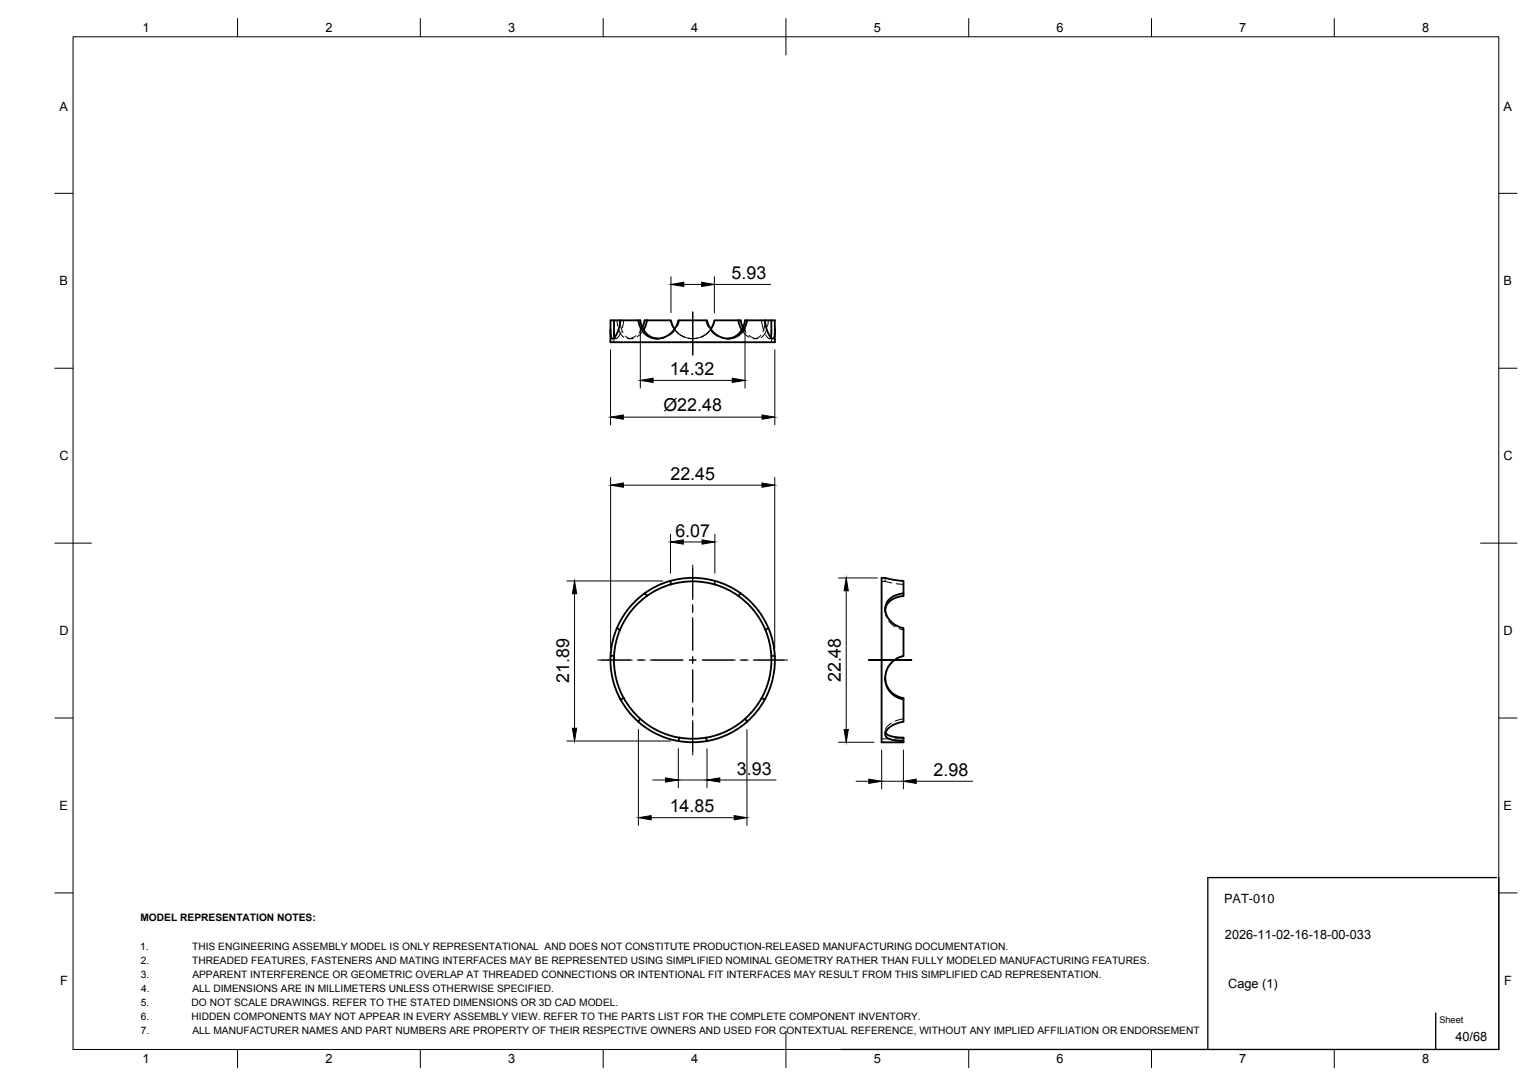
ISO-10303-21;
HEADER;
/* Generated by software containing ST-Developer
 * from STEP Tools, Inc. (www.steptools.com) 
 */

FILE_DESCRIPTION(
/* description */ ('Belt conveyor head drive unit'),
/* implementation_level */ '2;1');

FILE_NAME(
/* name */ 'Cage (1).step',
/* time_stamp */ '2026-10-28T03:26:19-07:00',
/* author */ (''),
/* organization */ (''),
/* preprocessor_version */ 'ST-DEVELOPER v20.2',
/* originating_system */ 'Autodesk Translation Framework v15.17.0.0',
/* authorisation */ '');

FILE_SCHEMA (('AUTOMOTIVE_DESIGN { 1 0 10303 214 3 1 1 }'));
ENDSEC;

DATA;
#10=MECHANICAL_DESIGN_GEOMETRIC_PRESENTATION_REPRESENTATION('',(#897),#27069);
#539=B_SPLINE_CURVE_WITH_KNOTS('',3,(#23163,#23164,#23165,#23166,#23167,
#23168,#23169,#23170,#23171,#23172,#23173,#23174,#23175,#23176,#23177,#23178,
#23179,#23180,#23181,#23182,#23183,#23184),.UNSPECIFIED.,.F.,.F.,(4,2,2,
2,2,2,2,2,2,2,4),(0.0591825211272536,0.157966726598481,0.236950089897721,
0.315933453196962,0.391576304923761,0.46721915665056,0.54286200837736,0.618504860104159,
0.697488223403399,0.77647158670264,0.875255792173867),.UNSPECIFIED.);
#540=B_SPLINE_CURVE_WITH_KNOTS('',3,(#23188,#23189,#23190,#23191,#23192,
#23193,#23194,#23195,#23196,#23197,#23198,#23199,#23200,#23201,#23202,#23203,
#23204,#23205,#23206,#23207,#23208,#23209),.UNSPECIFIED.,.F.,.F.,(4,2,2,
2,2,2,2,2,2,2,4),(0.0581119756758434,0.106553146291161,0.213106292582322,
0.30849933801665,0.386091982889075,0.4636846277615,0.541277272633925,0.61886991750635,
0.714262962940678,0.820816109231839,0.869257279847157),.UNSPECIFIED.);
#541=B_SPLINE_CURVE_WITH_KNOTS('',3,(#23215,#23216,#23217,#23218,#23219,
#23220,#23221,#23222,#23223,#23224,#23225,#23226,#23227,#23228,#23229,#23230,
#23231,#23232,#23233,#23234,#23235,#23236),.UNSPECIFIED.,.F.,.F.,(4,2,2,
2,2,2,2,2,2,2,4),(0.0581119756758434,0.106553146291161,0.213106292582322,
0.30849933801665,0.386091982889075,0.4636846277615,0.541277272633925,0.61886991750635,
0.714262962940679,0.820816109231839,0.869257279847157),.UNSPECIFIED.);
#542=B_SPLINE_CURVE_WITH_KNOTS('',3,(#23240,#23241,#23242,#23243,#23244,
#23245,#23246,#23247,#23248,#23249,#23250,#23251,#23252,#23253,#23254,#23255,
#23256,#23257,#23258,#23259,#23260,#23261),.UNSPECIFIED.,.F.,.F.,(4,2,2,
2,2,2,2,2,2,2,4),(0.0581119756758433,0.106553146291161,0.213106292582322,
0.308499338016649,0.386091982889075,0.4636846277615,0.541277272633925,0.61886991750635,
0.714262962940678,0.820816109231839,0.869257279847157),.UNSPECIFIED.);
#543=B_SPLINE_CURVE_WITH_KNOTS('',3,(#23270,#23271,#23272,#23273,#23274,
#23275,#23276,#23277,#23278,#23279,#23280,#23281,#23282,#23283,#23284,#23285,
#23286,#23287,#23288,#23289,#23290,#23291),.UNSPECIFIED.,.F.,.F.,(4,2,2,
2,2,2,2,2,2,2,4),(0.0581119756758433,0.106553146291161,0.213106292582322,
0.30849933801665,0.386091982889075,0.4636846277615,0.541277272633925,0.61886991750635,
0.714262962940678,0.820816109231839,0.869257279847157),.UNSPECIFIED.);
#544=B_SPLINE_CURVE_WITH_KNOTS('',3,(#23295,#23296,#23297,#23298,#23299,
#23300,#23301,#23302,#23303,#23304,#23305,#23306,#23307,#23308,#23309,#23310,
#23311,#23312,#23313,#23314,#23315,#23316),.UNSPECIFIED.,.F.,.F.,(4,2,2,
2,2,2,2,2,2,2,4),(0.0581119756758434,0.106553146291161,0.213106292582322,
0.30849933801665,0.386091982889075,0.4636846277615,0.541277272633925,0.61886991750635,
0.714262962940678,0.820816109231839,0.869257279847157),.UNSPECIFIED.);
#545=B_SPLINE_CURVE_WITH_KNOTS('',3,(#23320,#23321,#23322,#23323,#23324,
#23325,#23326,#23327,#23328,#23329,#23330,#23331,#23332,#23333,#23334,#23335,
#23336,#23337,#23338,#23339,#23340,#23341),.UNSPECIFIED.,.F.,.F.,(4,2,2,
2,2,2,2,2,2,2,4),(0.0581119756758434,0.106553146291161,0.213106292582322,
0.30849933801665,0.386091982889075,0.4636846277615,0.541277272633925,0.61886991750635,
0.714262962940678,0.820816109231839,0.869257279847157),.UNSPECIFIED.);
#546=B_SPLINE_CURVE_WITH_KNOTS('',3,(#23345,#23346,#23347,#23348,#23349,
#23350,#23351,#23352,#23353,#23354,#23355,#23356,#23357,#23358,#23359,#23360,
#23361,#23362,#23363,#23364,#23365,#23366),.UNSPECIFIED.,.F.,.F.,(4,2,2,
2,2,2,2,2,2,2,4),(0.0581119756758433,0.106553146291161,0.213106292582322,
0.30849933801665,0.386091982889075,0.4636846277615,0.541277272633925,0.61886991750635,
0.714262962940678,0.820816109231839,0.869257279847157),.UNSPECIFIED.);
#547=B_SPLINE_CURVE_WITH_KNOTS('',3,(#23374,#23375,#23376,#23377,#23378,
#23379,#23380,#23381,#23382,#23383,#23384,#23385,#23386,#23387,#23388,#23389,
#23390,#23391,#23392,#23393,#23394,#23395),.UNSPECIFIED.,.F.,.F.,(4,2,2,
2,2,2,2,2,2,2,4),(0.0591825211272536,0.157966726598481,0.236950089897721,
0.315933453196962,0.391576304923761,0.467219156650561,0.54286200837736,
0.618504860104159,0.697488223403399,0.77647158670264,0.875255792173867),
 .UNSPECIFIED.);
#548=B_SPLINE_CURVE_WITH_KNOTS('',3,(#23403,#23404,#23405,#23406,#23407,
#23408,#23409,#23410,#23411,#23412,#23413,#23414,#23415,#23416,#23417,#23418,
#23419,#23420,#23421,#23422,#23423,#23424),.UNSPECIFIED.,.F.,.F.,(4,2,2,
2,2,2,2,2,2,2,4),(0.0591825211272536,0.157966726598481,0.236950089897722,
0.315933453196962,0.391576304923761,0.467219156650561,0.54286200837736,
0.618504860104159,0.697488223403399,0.77647158670264,0.875255792173867),
 .UNSPECIFIED.);
#549=B_SPLINE_CURVE_WITH_KNOTS('',3,(#23434,#23435,#23436,#23437,#23438,
#23439,#23440,#23441,#23442,#23443,#23444,#23445,#23446,#23447,#23448,#23449,
#23450,#23451,#23452,#23453,#23454,#23455),.UNSPECIFIED.,.F.,.F.,(4,2,2,
2,2,2,2,2,2,2,4),(0.0591825211272536,0.157966726598481,0.236950089897721,
0.315933453196962,0.391576304923761,0.46721915665056,0.54286200837736,0.618504860104159,
0.697488223403399,0.77647158670264,0.875255792173867),.UNSPECIFIED.);
#550=B_SPLINE_CURVE_WITH_KNOTS('',3,(#23463,#23464,#23465,#23466,#23467,
#23468,#23469,#23470,#23471,#23472,#23473,#23474,#23475,#23476,#23477,#23478,
#23479,#23480,#23481,#23482,#23483,#23484),.UNSPECIFIED.,.F.,.F.,(4,2,2,
2,2,2,2,2,2,2,4),(0.0591825211272536,0.157966726598481,0.236950089897721,
0.315933453196962,0.391576304923761,0.46721915665056,0.542862008377359,
0.618504860104159,0.697488223403399,0.776471586702639,0.875255792173867),
 .UNSPECIFIED.);
#551=B_SPLINE_CURVE_WITH_KNOTS('',3,(#23492,#23493,#23494,#23495,#23496,
#23497,#23498,#23499,#23500,#23501,#23502,#23503,#23504,#23505,#23506,#23507,
#23508,#23509,#23510,#23511,#23512,#23513),.UNSPECIFIED.,.F.,.F.,(4,2,2,
2,2,2,2,2,2,2,4),(0.0591825211272536,0.157966726598481,0.236950089897721,
0.315933453196962,0.391576304923761,0.46721915665056,0.54286200837736,0.618504860104159,
0.697488223403399,0.77647158670264,0.875255792173867),.UNSPECIFIED.);
#552=B_SPLINE_CURVE_WITH_KNOTS('',3,(#23522,#23523,#23524,#23525,#23526,
#23527,#23528,#23529,#23530,#23531,#23532,#23533,#23534,#23535,#23536,#23537,
#23538,#23539,#23540,#23541,#23542,#23543),.UNSPECIFIED.,.F.,.F.,(4,2,2,
2,2,2,2,2,2,2,4),(0.0591825211272536,0.157966726598481,0.236950089897721,
0.315933453196962,0.391576304923761,0.46721915665056,0.542862008377359,
0.618504860104159,0.697488223403399,0.776471586702639,0.875255792173867),
 .UNSPECIFIED.);
#668=SPHERICAL_SURFACE('',#15410,0.309556);
#669=SPHERICAL_SURFACE('',#15426,0.309556);
#670=SPHERICAL_SURFACE('',#15431,0.309556);
#671=SPHERICAL_SURFACE('',#15437,0.309556);
#672=SPHERICAL_SURFACE('',#15442,0.309556);
#673=SPHERICAL_SURFACE('',#15447,0.309556);
#674=SPHERICAL_SURFACE('',#15455,0.309556);
#745=SHAPE_REPRESENTATION_RELATIONSHIP('SRR','None',#27391,#814);
#814=ADVANCED_BREP_SHAPE_REPRESENTATION('',(#981),#27033);
#897=STYLED_ITEM('',(#27797),#981);
#981=MANIFOLD_SOLID_BREP('Continuous crown cage',#13763);
#1166=FACE_BOUND('',#2998,.T.);
#1470=PLANE('',#15423);
#1471=PLANE('',#15428);
#1472=PLANE('',#15433);
#1473=PLANE('',#15439);
#1474=PLANE('',#15444);
#1475=PLANE('',#15453);
#1476=PLANE('',#15457);
#1477=PLANE('',#15458);
#2028=FACE_OUTER_BOUND('',#2982,.T.);
#2029=FACE_OUTER_BOUND('',#2983,.T.);
#2030=FACE_OUTER_BOUND('',#2984,.T.);
#2031=FACE_OUTER_BOUND('',#2985,.T.);
#2032=FACE_OUTER_BOUND('',#2986,.T.);
#2033=FACE_OUTER_BOUND('',#2987,.T.);
#2034=FACE_OUTER_BOUND('',#2988,.T.);
#2035=FACE_OUTER_BOUND('',#2989,.T.);
#2036=FACE_OUTER_BOUND('',#2990,.T.);
#2037=FACE_OUTER_BOUND('',#2991,.T.);
#2038=FACE_OUTER_BOUND('',#2992,.T.);
#2039=FACE_OUTER_BOUND('',#2993,.T.);
#2040=FACE_OUTER_BOUND('',#2994,.T.);
#2041=FACE_OUTER_BOUND('',#2995,.T.);
#2042=FACE_OUTER_BOUND('',#2996,.T.);
#2043=FACE_OUTER_BOUND('',#2997,.T.);
#2044=FACE_OUTER_BOUND('',#2999,.T.);
#2982=EDGE_LOOP('',(#10632,#10633,#10634,#10635));
#2983=EDGE_LOOP('',(#10636,#10637,#10638,#10639,#10640,#10641,#10642,#10643,
#10644,#10645,#10646,#10647,#10648,#10649,#10650,#10651,#10652,#10653));
#2984=EDGE_LOOP('',(#10654,#10655,#10656,#10657));
#2985=EDGE_LOOP('',(#10658,#10659,#10660,#10661));
#2986=EDGE_LOOP('',(#10662,#10663,#10664,#10665));
#2987=EDGE_LOOP('',(#10666,#10667,#10668,#10669));
#2988=EDGE_LOOP('',(#10670,#10671,#10672,#10673,#10674,#10675));
#2989=EDGE_LOOP('',(#10676,#10677,#10678,#10679));
#2990=EDGE_LOOP('',(#10680,#10681,#10682,#10683));
#2991=EDGE_LOOP('',(#10684,#10685,#10686,#10687));
#2992=EDGE_LOOP('',(#10688,#10689,#10690,#10691));
#2993=EDGE_LOOP('',(#10692,#10693,#10694,#10695));
#2994=EDGE_LOOP('',(#10696,#10697,#10698,#10699,#10700,#10701,#10702,#10703,
#10704,#10705,#10706,#10707,#10708,#10709,#10710,#10711,#10712,#10713));
#2995=EDGE_LOOP('',(#10714,#10715,#10716,#10717));
#2996=EDGE_LOOP('',(#10718,#10719,#10720,#10721));
#2997=EDGE_LOOP('',(#10722));
#2998=EDGE_LOOP('',(#10723));
#2999=EDGE_LOOP('',(#10724,#10725,#10726,#10727));
#3910=LINE('',#23265,#4702);
#3911=LINE('',#23518,#4703);
#4702=VECTOR('',#18556,1.123812);
#4703=VECTOR('',#18625,1.076188);
#5489=CIRCLE('',#15411,0.303778037777585);
#5490=CIRCLE('',#15412,0.303778037777585);
#5491=CIRCLE('',#15414,1.123812);
#5492=CIRCLE('',#15415,1.123812);
#5493=CIRCLE('',#15416,1.123812);
#5494=CIRCLE('',#15417,1.123812);
#5495=CIRCLE('',#15418,1.123812);
#5496=CIRCLE('',#15419,1.123812);
#5497=CIRCLE('',#15420,1.123812);
#5498=CIRCLE('',#15421,1.123812);
#5499=CIRCLE('',#15422,1.123812);
#5500=CIRCLE('',#15424,1.076188);
#5501=CIRCLE('',#15425,0.303778037777585);
#5502=CIRCLE('',#15427,0.303778037777585);
#5503=CIRCLE('',#15429,1.076188);
#5504=CIRCLE('',#15430,0.303778037777585);
#5505=CIRCLE('',#15432,0.303778037777585);
#5506=CIRCLE('',#15434,1.076188);
#5507=CIRCLE('',#15435,1.076188);
#5508=CIRCLE('',#15436,0.303778037777585);
#5509=CIRCLE('',#15438,0.303778037777585);
#5510=CIRCLE('',#15440,1.076188);
#5511=CIRCLE('',#15441,0.303778037777585);
#5512=CIRCLE('',#15443,0.303778037777585);
#5513=CIRCLE('',#15445,1.076188);
#5514=CIRCLE('',#15446,0.303778037777585);
#5515=CIRCLE('',#15448,0.303778037777585);
#5516=CIRCLE('',#15450,1.076188);
#5517=CIRCLE('',#15451,1.076188);
#5518=CIRCLE('',#15452,1.076188);
#5519=CIRCLE('',#15454,0.303778037777585);
#5520=CIRCLE('',#15456,0.303778037777585);
#6527=VERTEX_POINT('',#23161);
#6528=VERTEX_POINT('',#23162);
#6529=VERTEX_POINT('',#23185);
#6530=VERTEX_POINT('',#23187);
#6531=VERTEX_POINT('',#23212);
#6532=VERTEX_POINT('',#23214);
#6533=VERTEX_POINT('',#23237);
#6534=VERTEX_POINT('',#23239);
#6535=VERTEX_POINT('',#23262);
#6536=VERTEX_POINT('',#23264);
#6537=VERTEX_POINT('',#23267);
#6538=VERTEX_POINT('',#23269);
#6539=VERTEX_POINT('',#23292);
#6540=VERTEX_POINT('',#23294);
#6541=VERTEX_POINT('',#23317);
#6542=VERTEX_POINT('',#23319);
#6543=VERTEX_POINT('',#23342);
#6544=VERTEX_POINT('',#23344);
#6545=VERTEX_POINT('',#23369);
#6546=VERTEX_POINT('',#23373);
#6547=VERTEX_POINT('',#23398);
#6548=VERTEX_POINT('',#23402);
#6549=VERTEX_POINT('',#23427);
#6550=VERTEX_POINT('',#23429);
#6551=VERTEX_POINT('',#23433);
#6552=VERTEX_POINT('',#23458);
#6553=VERTEX_POINT('',#23462);
#6554=VERTEX_POINT('',#23487);
#6555=VERTEX_POINT('',#23491);
#6556=VERTEX_POINT('',#23516);
#6557=VERTEX_POINT('',#23519);
#6558=VERTEX_POINT('',#23521);
#8008=EDGE_CURVE('',#6527,#6528,#539,.T.);
#8009=EDGE_CURVE('',#6529,#6527,#5489,.T.);
#8010=EDGE_CURVE('',#6530,#6529,#540,.T.);
#8011=EDGE_CURVE('',#6528,#6530,#5490,.T.);
#8012=EDGE_CURVE('',#6531,#6529,#5491,.T.);
#8013=EDGE_CURVE('',#6531,#6532,#541,.T.);
#8014=EDGE_CURVE('',#6533,#6532,#5492,.T.);
#8015=EDGE_CURVE('',#6533,#6534,#542,.T.);
#8016=EDGE_CURVE('',#6535,#6534,#5493,.T.);
#8017=EDGE_CURVE('',#6535,#6536,#3910,.T.);
#8018=EDGE_CURVE('',#6536,#6536,#5494,.T.);
#8019=EDGE_CURVE('',#6537,#6535,#5495,.T.);
#8020=EDGE_CURVE('',#6537,#6538,#543,.T.);
#8021=EDGE_CURVE('',#6539,#6538,#5496,.T.);
#8022=EDGE_CURVE('',#6539,#6540,#544,.T.);
#8023=EDGE_CURVE('',#6541,#6540,#5497,.T.);
#8024=EDGE_CURVE('',#6541,#6542,#545,.T.);
#8025=EDGE_CURVE('',#6543,#6542,#5498,.T.);
#8026=EDGE_CURVE('',#6543,#6544,#546,.T.);
#8027=EDGE_CURVE('',#6530,#6544,#5499,.T.);
#8028=EDGE_CURVE('',#6527,#6545,#5500,.T.);
#8029=EDGE_CURVE('',#6545,#6531,#5501,.T.);
#8030=EDGE_CURVE('',#6546,#6545,#547,.T.);
#8031=EDGE_CURVE('',#6532,#6546,#5502,.T.);
#8032=EDGE_CURVE('',#6546,#6547,#5503,.T.);
#8033=EDGE_CURVE('',#6547,#6533,#5504,.T.);
#8034=EDGE_CURVE('',#6548,#6547,#548,.T.);
#8035=EDGE_CURVE('',#6534,#6548,#5505,.T.);
#8036=EDGE_CURVE('',#6548,#6549,#5506,.T.);
#8037=EDGE_CURVE('',#6549,#6550,#5507,.T.);
#8038=EDGE_CURVE('',#6550,#6537,#5508,.T.);
#8039=EDGE_CURVE('',#6551,#6550,#549,.T.);
#8040=EDGE_CURVE('',#6538,#6551,#5509,.T.);
#8041=EDGE_CURVE('',#6551,#6552,#5510,.T.);
#8042=EDGE_CURVE('',#6552,#6539,#5511,.T.);
#8043=EDGE_CURVE('',#6553,#6552,#550,.T.);
#8044=EDGE_CURVE('',#6540,#6553,#5512,.T.);
#8045=EDGE_CURVE('',#6553,#6554,#5513,.T.);
#8046=EDGE_CURVE('',#6554,#6541,#5514,.T.);
#8047=EDGE_CURVE('',#6555,#6554,#551,.T.);
#8048=EDGE_CURVE('',#6542,#6555,#5515,.T.);
#8049=EDGE_CURVE('',#6556,#6556,#5516,.T.);
#8050=EDGE_CURVE('',#6556,#6549,#3911,.T.);
#8051=EDGE_CURVE('',#6557,#6528,#5517,.T.);
#8052=EDGE_CURVE('',#6557,#6558,#552,.T.);
#8053=EDGE_CURVE('',#6555,#6558,#5518,.T.);
#8054=EDGE_CURVE('',#6544,#6557,#5519,.T.);
#8055=EDGE_CURVE('',#6558,#6543,#5520,.T.);
#10632=ORIENTED_EDGE('',*,*,#8008,.F.);
#10633=ORIENTED_EDGE('',*,*,#8009,.F.);
#10634=ORIENTED_EDGE('',*,*,#8010,.F.);
#10635=ORIENTED_EDGE('',*,*,#8011,.F.);
#10636=ORIENTED_EDGE('',*,*,#8010,.T.);
#10637=ORIENTED_EDGE('',*,*,#8012,.F.);
#10638=ORIENTED_EDGE('',*,*,#8013,.T.);
#10639=ORIENTED_EDGE('',*,*,#8014,.F.);
#10640=ORIENTED_EDGE('',*,*,#8015,.T.);
#10641=ORIENTED_EDGE('',*,*,#8016,.F.);
#10642=ORIENTED_EDGE('',*,*,#8017,.T.);
#10643=ORIENTED_EDGE('',*,*,#8018,.F.);
#10644=ORIENTED_EDGE('',*,*,#8017,.F.);
#10645=ORIENTED_EDGE('',*,*,#8019,.F.);
#10646=ORIENTED_EDGE('',*,*,#8020,.T.);
#10647=ORIENTED_EDGE('',*,*,#8021,.F.);
#10648=ORIENTED_EDGE('',*,*,#8022,.T.);
#10649=ORIENTED_EDGE('',*,*,#8023,.F.);
#10650=ORIENTED_EDGE('',*,*,#8024,.T.);
#10651=ORIENTED_EDGE('',*,*,#8025,.F.);
#10652=ORIENTED_EDGE('',*,*,#8026,.T.);
#10653=ORIENTED_EDGE('',*,*,#8027,.F.);
#10654=ORIENTED_EDGE('',*,*,#8009,.T.);
#10655=ORIENTED_EDGE('',*,*,#8028,.T.);
#10656=ORIENTED_EDGE('',*,*,#8029,.T.);
#10657=ORIENTED_EDGE('',*,*,#8012,.T.);
#10658=ORIENTED_EDGE('',*,*,#8030,.F.);
#10659=ORIENTED_EDGE('',*,*,#8031,.F.);
#10660=ORIENTED_EDGE('',*,*,#8013,.F.);
#10661=ORIENTED_EDGE('',*,*,#8029,.F.);
#10662=ORIENTED_EDGE('',*,*,#8031,.T.);
#10663=ORIENTED_EDGE('',*,*,#8032,.T.);
#10664=ORIENTED_EDGE('',*,*,#8033,.T.);
#10665=ORIENTED_EDGE('',*,*,#8014,.T.);
#10666=ORIENTED_EDGE('',*,*,#8034,.F.);
#10667=ORIENTED_EDGE('',*,*,#8035,.F.);
#10668=ORIENTED_EDGE('',*,*,#8015,.F.);
#10669=ORIENTED_EDGE('',*,*,#8033,.F.);
#10670=ORIENTED_EDGE('',*,*,#8035,.T.);
#10671=ORIENTED_EDGE('',*,*,#8036,.T.);
#10672=ORIENTED_EDGE('',*,*,#8037,.T.);
#10673=ORIENTED_EDGE('',*,*,#8038,.T.);
#10674=ORIENTED_EDGE('',*,*,#8019,.T.);
#10675=ORIENTED_EDGE('',*,*,#8016,.T.);
#10676=ORIENTED_EDGE('',*,*,#8039,.F.);
#10677=ORIENTED_EDGE('',*,*,#8040,.F.);
#10678=ORIENTED_EDGE('',*,*,#8020,.F.);
#10679=ORIENTED_EDGE('',*,*,#8038,.F.);
#10680=ORIENTED_EDGE('',*,*,#8040,.T.);
#10681=ORIENTED_EDGE('',*,*,#8041,.T.);
#10682=ORIENTED_EDGE('',*,*,#8042,.T.);
#10683=ORIENTED_EDGE('',*,*,#8021,.T.);
#10684=ORIENTED_EDGE('',*,*,#8043,.F.);
#10685=ORIENTED_EDGE('',*,*,#8044,.F.);
#10686=ORIENTED_EDGE('',*,*,#8022,.F.);
#10687=ORIENTED_EDGE('',*,*,#8042,.F.);
#10688=ORIENTED_EDGE('',*,*,#8044,.T.);
#10689=ORIENTED_EDGE('',*,*,#8045,.T.);
#10690=ORIENTED_EDGE('',*,*,#8046,.T.);
#10691=ORIENTED_EDGE('',*,*,#8023,.T.);
#10692=ORIENTED_EDGE('',*,*,#8024,.F.);
#10693=ORIENTED_EDGE('',*,*,#8046,.F.);
#10694=ORIENTED_EDGE('',*,*,#8047,.F.);
#10695=ORIENTED_EDGE('',*,*,#8048,.F.);
#10696=ORIENTED_EDGE('',*,*,#8049,.F.);
#10697=ORIENTED_EDGE('',*,*,#8050,.T.);
#10698=ORIENTED_EDGE('',*,*,#8036,.F.);
#10699=ORIENTED_EDGE('',*,*,#8034,.T.);
#10700=ORIENTED_EDGE('',*,*,#8032,.F.);
#10701=ORIENTED_EDGE('',*,*,#8030,.T.);
#10702=ORIENTED_EDGE('',*,*,#8028,.F.);
#10703=ORIENTED_EDGE('',*,*,#8008,.T.);
#10704=ORIENTED_EDGE('',*,*,#8051,.F.);
#10705=ORIENTED_EDGE('',*,*,#8052,.T.);
#10706=ORIENTED_EDGE('',*,*,#8053,.F.);
#10707=ORIENTED_EDGE('',*,*,#8047,.T.);
#10708=ORIENTED_EDGE('',*,*,#8045,.F.);
#10709=ORIENTED_EDGE('',*,*,#8043,.T.);
#10710=ORIENTED_EDGE('',*,*,#8041,.F.);
#10711=ORIENTED_EDGE('',*,*,#8039,.T.);
#10712=ORIENTED_EDGE('',*,*,#8037,.F.);
#10713=ORIENTED_EDGE('',*,*,#8050,.F.);
#10714=ORIENTED_EDGE('',*,*,#8011,.T.);
#10715=ORIENTED_EDGE('',*,*,#8027,.T.);
#10716=ORIENTED_EDGE('',*,*,#8054,.T.);
#10717=ORIENTED_EDGE('',*,*,#8051,.T.);
#10718=ORIENTED_EDGE('',*,*,#8026,.F.);
#10719=ORIENTED_EDGE('',*,*,#8055,.F.);
#10720=ORIENTED_EDGE('',*,*,#8052,.F.);
#10721=ORIENTED_EDGE('',*,*,#8054,.F.);
#10722=ORIENTED_EDGE('',*,*,#8018,.T.);
#10723=ORIENTED_EDGE('',*,*,#8049,.T.);
#10724=ORIENTED_EDGE('',*,*,#8048,.T.);
#10725=ORIENTED_EDGE('',*,*,#8053,.T.);
#10726=ORIENTED_EDGE('',*,*,#8055,.T.);
#10727=ORIENTED_EDGE('',*,*,#8025,.T.);
#12695=CYLINDRICAL_SURFACE('',#15413,1.123812);
#12696=CYLINDRICAL_SURFACE('',#15449,1.076188);
#13307=ADVANCED_FACE('',(#2028),#668,.F.);
#13308=ADVANCED_FACE('',(#2029),#12695,.T.);
#13309=ADVANCED_FACE('',(#2030),#1470,.T.);
#13310=ADVANCED_FACE('',(#2031),#669,.F.);
#13311=ADVANCED_FACE('',(#2032),#1471,.T.);
#13312=ADVANCED_FACE('',(#2033),#670,.F.);
#13313=ADVANCED_FACE('',(#2034),#1472,.T.);
#13314=ADVANCED_FACE('',(#2035),#671,.F.);
#13315=ADVANCED_FACE('',(#2036),#1473,.T.);
#13316=ADVANCED_FACE('',(#2037),#672,.F.);
#13317=ADVANCED_FACE('',(#2038),#1474,.T.);
#13318=ADVANCED_FACE('',(#2039),#673,.F.);
#13319=ADVANCED_FACE('',(#2040),#12696,.F.);
#13320=ADVANCED_FACE('',(#2041),#1475,.T.);
#13321=ADVANCED_FACE('',(#2042),#674,.F.);
#13322=ADVANCED_FACE('',(#2043,#1166),#1476,.T.);
#13323=ADVANCED_FACE('',(#2044),#1477,.T.);
#13763=CLOSED_SHELL('',(#13307,#13308,#13309,#13310,#13311,#13312,#13313,
#13314,#13315,#13316,#13317,#13318,#13319,#13320,#13321,#13322,#13323));
#15409=AXIS2_PLACEMENT_3D('',#23159,#18540,#18541);
#15410=AXIS2_PLACEMENT_3D('',#23160,#18542,#18543);
#15411=AXIS2_PLACEMENT_3D('',#23186,#18544,#18545);
#15412=AXIS2_PLACEMENT_3D('',#23210,#18546,#18547);
#15413=AXIS2_PLACEMENT_3D('',#23211,#18548,#18549);
#15414=AXIS2_PLACEMENT_3D('',#23213,#18550,#18551);
#15415=AXIS2_PLACEMENT_3D('',#23238,#18552,#18553);
#15416=AXIS2_PLACEMENT_3D('',#23263,#18554,#18555);
#15417=AXIS2_PLACEMENT_3D('',#23266,#18557,#18558);
#15418=AXIS2_PLACEMENT_3D('',#23268,#18559,#18560);
#15419=AXIS2_PLACEMENT_3D('',#23293,#18561,#18562);
#15420=AXIS2_PLACEMENT_3D('',#23318,#18563,#18564);
#15421=AXIS2_PLACEMENT_3D('',#23343,#18565,#18566);
#15422=AXIS2_PLACEMENT_3D('',#23367,#18567,#18568);
#15423=AXIS2_PLACEMENT_3D('',#23368,#18569,#18570);
#15424=AXIS2_PLACEMENT_3D('',#23370,#18571,#18572);
#15425=AXIS2_PLACEMENT_3D('',#23371,#18573,#18574);
#15426=AXIS2_PLACEMENT_3D('',#23372,#18575,#18576);
#15427=AXIS2_PLACEMENT_3D('',#23396,#18577,#18578);
#15428=AXIS2_PLACEMENT_3D('',#23397,#18579,#18580);
#15429=AXIS2_PLACEMENT_3D('',#23399,#18581,#18582);
#15430=AXIS2_PLACEMENT_3D('',#23400,#18583,#18584);
#15431=AXIS2_PLACEMENT_3D('',#23401,#18585,#18586);
#15432=AXIS2_PLACEMENT_3D('',#23425,#18587,#18588);
#15433=AXIS2_PLACEMENT_3D('',#23426,#18589,#18590);
#15434=AXIS2_PLACEMENT_3D('',#23428,#18591,#18592);
#15435=AXIS2_PLACEMENT_3D('',#23430,#18593,#18594);
#15436=AXIS2_PLACEMENT_3D('',#23431,#18595,#18596);
#15437=AXIS2_PLACEMENT_3D('',#23432,#18597,#18598);
#15438=AXIS2_PLACEMENT_3D('',#23456,#18599,#18600);
#15439=AXIS2_PLACEMENT_3D('',#23457,#18601,#18602);
#15440=AXIS2_PLACEMENT_3D('',#23459,#18603,#18604);
#15441=AXIS2_PLACEMENT_3D('',#23460,#18605,#18606);
#15442=AXIS2_PLACEMENT_3D('',#23461,#18607,#18608);
#15443=AXIS2_PLACEMENT_3D('',#23485,#18609,#18610);
#15444=AXIS2_PLACEMENT_3D('',#23486,#18611,#18612);
#15445=AXIS2_PLACEMENT_3D('',#23488,#18613,#18614);
#15446=AXIS2_PLACEMENT_3D('',#23489,#18615,#18616);
#15447=AXIS2_PLACEMENT_3D('',#23490,#18617,#18618);
#15448=AXIS2_PLACEMENT_3D('',#23514,#18619,#18620);
#15449=AXIS2_PLACEMENT_3D('',#23515,#18621,#18622);
#15450=AXIS2_PLACEMENT_3D('',#23517,#18623,#18624);
#15451=AXIS2_PLACEMENT_3D('',#23520,#18626,#18627);
#15452=AXIS2_PLACEMENT_3D('',#23544,#18628,#18629);
#15453=AXIS2_PLACEMENT_3D('',#23545,#18630,#18631);
#15454=AXIS2_PLACEMENT_3D('',#23546,#18632,#18633);
#15455=AXIS2_PLACEMENT_3D('',#23547,#18634,#18635);
#15456=AXIS2_PLACEMENT_3D('',#23548,#18636,#18637);
#15457=AXIS2_PLACEMENT_3D('',#23549,#18638,#18639);
#15458=AXIS2_PLACEMENT_3D('',#23550,#18640,#18641);
#18540=DIRECTION('axis',(0.,0.,1.));
#18541=DIRECTION('refdir',(1.,0.,0.));
#18542=DIRECTION('center_axis',(0.,0.,1.));
#18543=DIRECTION('ref_axis',(1.,0.,0.));
#18544=DIRECTION('center_axis',(0.,-1.,0.));
#18545=DIRECTION('ref_axis',(0.,0.,-1.));
#18546=DIRECTION('center_axis',(0.,-1.,0.));
#18547=DIRECTION('ref_axis',(0.,0.,-1.));
#18548=DIRECTION('center_axis',(0.,1.,0.));
#18549=DIRECTION('ref_axis',(1.,0.,0.));
#18550=DIRECTION('center_axis',(0.,1.,0.));
#18551=DIRECTION('ref_axis',(1.,0.,0.));
#18552=DIRECTION('center_axis',(0.,1.,0.));
#18553=DIRECTION('ref_axis',(1.,0.,0.));
#18554=DIRECTION('center_axis',(0.,1.,0.));
#18555=DIRECTION('ref_axis',(1.,0.,0.));
#18556=DIRECTION('',(0.,-1.,0.));
#18557=DIRECTION('center_axis',(0.,-1.,0.));
#18558=DIRECTION('ref_axis',(1.,0.,0.));
#18559=DIRECTION('center_axis',(0.,1.,0.));
#18560=DIRECTION('ref_axis',(1.,0.,0.));
#18561=DIRECTION('center_axis',(0.,1.,0.));
#18562=DIRECTION('ref_axis',(1.,0.,0.));
#18563=DIRECTION('center_axis',(0.,1.,0.));
#18564=DIRECTION('ref_axis',(1.,0.,0.));
#18565=DIRECTION('center_axis',(0.,1.,0.));
#18566=DIRECTION('ref_axis',(1.,0.,0.));
#18567=DIRECTION('center_axis',(0.,1.,0.));
#18568=DIRECTION('ref_axis',(1.,0.,0.));
#18569=DIRECTION('center_axis',(0.,1.,0.));
#18570=DIRECTION('ref_axis',(1.,0.,0.));
#18571=DIRECTION('center_axis',(0.,-1.,0.));
#18572=DIRECTION('ref_axis',(1.,0.,0.));
#18573=DIRECTION('center_axis',(0.,-1.,0.));
#18574=DIRECTION('ref_axis',(0.,0.,-1.));
#18575=DIRECTION('center_axis',(8.96625347776458E-17,0.,1.));
#18576=DIRECTION('ref_axis',(1.,0.,0.));
#18577=DIRECTION('center_axis',(0.,-1.,0.));
#18578=DIRECTION('ref_axis',(0.,0.,-1.));
#18579=DIRECTION('center_axis',(0.,1.,0.));
#18580=DIRECTION('ref_axis',(1.,0.,0.));
#18581=DIRECTION('center_axis',(0.,-1.,0.));
#18582=DIRECTION('ref_axis',(1.,0.,0.));
#18583=DIRECTION('center_axis',(0.,-1.,0.));
#18584=DIRECTION('ref_axis',(0.,0.,-1.));
#18585=DIRECTION('center_axis',(0.,0.,1.));
#18586=DIRECTION('ref_axis',(1.,0.,0.));
#18587=DIRECTION('center_axis',(0.,-1.,0.));
#18588=DIRECTION('ref_axis',(0.,0.,-1.));
#18589=DIRECTION('center_axis',(0.,1.,0.));
#18590=DIRECTION('ref_axis',(1.,0.,0.));
#18591=DIRECTION('center_axis',(0.,-1.,0.));
#18592=DIRECTION('ref_axis',(1.,0.,0.));
#18593=DIRECTION('center_axis',(0.,-1.,0.));
#18594=DIRECTION('ref_axis',(1.,0.,0.));
#18595=DIRECTION('center_axis',(0.,-1.,0.));
#18596=DIRECTION('ref_axis',(0.,0.,-1.));
#18597=DIRECTION('center_axis',(0.,0.,1.));
#18598=DIRECTION('ref_axis',(1.,0.,0.));
#18599=DIRECTION('center_axis',(0.,-1.,0.));
#18600=DIRECTION('ref_axis',(0.,0.,-1.));
#18601=DIRECTION('center_axis',(0.,1.,0.));
#18602=DIRECTION('ref_axis',(1.,0.,0.));
#18603=DIRECTION('center_axis',(0.,-1.,0.));
#18604=DIRECTION('ref_axis',(1.,0.,0.));
#18605=DIRECTION('center_axis',(0.,-1.,0.));
#18606=DIRECTION('ref_axis',(0.,0.,-1.));
#18607=DIRECTION('center_axis',(8.96625347776458E-17,0.,1.));
#18608=DIRECTION('ref_axis',(1.,0.,0.));
#18609=DIRECTION('center_axis',(0.,-1.,0.));
#18610=DIRECTION('ref_axis',(0.,0.,-1.));
#18611=DIRECTION('center_axis',(0.,1.,0.));
#18612=DIRECTION('ref_axis',(1.,0.,0.));
#18613=DIRECTION('center_axis',(0.,-1.,0.));
#18614=DIRECTION('ref_axis',(1.,0.,0.));
#18615=DIRECTION('center_axis',(0.,-1.,0.));
#18616=DIRECTION('ref_axis',(0.,0.,-1.));
#18617=DIRECTION('center_axis',(0.,0.,1.));
#18618=DIRECTION('ref_axis',(1.,0.,0.));
#18619=DIRECTION('center_axis',(0.,-1.,0.));
#18620=DIRECTION('ref_axis',(0.,0.,-1.));
#18621=DIRECTION('center_axis',(0.,1.,0.));
#18622=DIRECTION('ref_axis',(1.,0.,0.));
#18623=DIRECTION('center_axis',(0.,1.,0.));
#18624=DIRECTION('ref_axis',(1.,0.,0.));
#18625=DIRECTION('',(0.,1.,0.));
#18626=DIRECTION('center_axis',(0.,-1.,0.));
#18627=DIRECTION('ref_axis',(1.,0.,0.));
#18628=DIRECTION('center_axis',(0.,-1.,0.));
#18629=DIRECTION('ref_axis',(1.,0.,0.));
#18630=DIRECTION('center_axis',(0.,1.,0.));
#18631=DIRECTION('ref_axis',(1.,0.,0.));
#18632=DIRECTION('center_axis',(0.,-1.,0.));
#18633=DIRECTION('ref_axis',(0.,0.,-1.));
#18634=DIRECTION('center_axis',(0.,0.,1.));
#18635=DIRECTION('ref_axis',(1.,0.,0.));
#18636=DIRECTION('center_axis',(0.,-1.,0.));
#18637=DIRECTION('ref_axis',(0.,0.,-1.));
#18638=DIRECTION('center_axis',(0.,-1.,0.));
#18639=DIRECTION('ref_axis',(-1.,0.,0.));
#18640=DIRECTION('center_axis',(0.,1.,0.));
#18641=DIRECTION('ref_axis',(1.,0.,0.));
#23159=CARTESIAN_POINT('',(0.,0.,0.));
#23160=CARTESIAN_POINT('Origin',(0.685838782044607,0.,0.860014630714833));
#23161=CARTESIAN_POINT('',(0.413083465285518,-0.05953,0.993751811093549));
#23162=CARTESIAN_POINT('',(0.876916659919095,-0.05953,0.623857181492959));
#23163=CARTESIAN_POINT('Ctrl Pts',(0.413083465285518,-0.05953,0.993751811093549));
#23164=CARTESIAN_POINT('Ctrl Pts',(0.419070565453383,-0.0925528133349865,
0.991263089003441));
#23165=CARTESIAN_POINT('Ctrl Pts',(0.430199341854858,-0.124911173756694,
0.986608710139579));
#23166=CARTESIAN_POINT('Ctrl Pts',(0.457978755888596,-0.177924977804098,
0.973971221090534));
#23167=CARTESIAN_POINT('Ctrl Pts',(0.473077587363685,-0.199697230012983,
0.966820759530997));
#23168=CARTESIAN_POINT('Ctrl Pts',(0.507057380724533,-0.237895043532788,
0.949440676105255));
#23169=CARTESIAN_POINT('Ctrl Pts',(0.525933334162555,-0.254319232363049,
0.939198248544428));
#23170=CARTESIAN_POINT('Ctrl Pts',(0.564362943424238,-0.28018331644634,
0.916597376014514));
#23171=CARTESIAN_POINT('Ctrl Pts',(0.585840553788742,-0.29104845371857,
0.903141581680914));
#23172=CARTESIAN_POINT('Ctrl Pts',(0.629305439856167,-0.30527573347708,
0.873412008702649));
#23173=CARTESIAN_POINT('Ctrl Pts',(0.651278921914856,-0.308638795020976,
0.857118508332695));
#23174=CARTESIAN_POINT('Ctrl Pts',(0.690705563850638,-0.308638795020976,
0.825676810575914));
#23175=CARTESIAN_POINT('Ctrl Pts',(0.711480111898423,-0.30527573347708,
0.807879894508811));
#23176=CARTESIAN_POINT('Ctrl Pts',(0.750136149454208,-0.29104845371857,
0.772120216227122));
#23177=CARTESIAN_POINT('Ctrl Pts',(0.768033796848072,-0.28018331644634,
0.754175290318038));
#23178=CARTESIAN_POINT('Ctrl Pts',(0.798619410861634,-0.254319232363049,
0.721738358858166));
#23179=CARTESIAN_POINT('Ctrl Pts',(0.812805334167529,-0.237895043532788,
0.705614819529209));
#23180=CARTESIAN_POINT('Ctrl Pts',(0.837310877969633,-0.199697230012983,
0.676354402927683));
#23181=CARTESIAN_POINT('Ctrl Pts',(0.847641868610495,-0.177924977804098,
0.663225258065736));
#23182=CARTESIAN_POINT('Ctrl Pts',(0.866144010579847,-0.124911173756694,
0.638954437806245));
#23183=CARTESIAN_POINT('Ctrl Pts',(0.873158080166742,-0.0925528133349865,
0.62914037979579));
#23184=CARTESIAN_POINT('Ctrl Pts',(0.876916659919095,-0.05953,0.623857181492959));
#23185=CARTESIAN_POINT('',(0.437601487681057,-0.05953,1.03511272300331));
#23186=CARTESIAN_POINT('Origin',(0.685838782044607,-0.05953,0.860014630714833));
#23187=CARTESIAN_POINT('',(0.911784794170997,-0.05953,0.656964154625313));
#23188=CARTESIAN_POINT('Ctrl Pts',(0.911784794170998,-0.0595300000000001,
0.656964154625312));
#23189=CARTESIAN_POINT('Ctrl Pts',(0.909827729890942,-0.0762225747374255,
0.659680317203144));
#23190=CARTESIAN_POINT('Ctrl Pts',(0.907004864562642,-0.0928409665394228,
0.663576540841106));
#23191=CARTESIAN_POINT('Ctrl Pts',(0.895234408667242,-0.144299303100741,
0.679480524217551));
#23192=CARTESIAN_POINT('Ctrl Pts',(0.882797231409153,-0.177024326825049,
0.695831250979106));
#23193=CARTESIAN_POINT('Ctrl Pts',(0.854332839576145,-0.227269801620064,
0.73042219438957));
#23194=CARTESIAN_POINT('Ctrl Pts',(0.834863020612702,-0.251265615809407,
0.752807465209441));
#23195=CARTESIAN_POINT('Ctrl Pts',(0.800439809856111,-0.279889827963178,
0.789147407129766));
#23196=CARTESIAN_POINT('Ctrl Pts',(0.781998747691871,-0.290879136862659,
0.80756613568454));
#23197=CARTESIAN_POINT('Ctrl Pts',(0.742239891936898,-0.305251990234487,
0.844254137480382));
#23198=CARTESIAN_POINT('Ctrl Pts',(0.720906778729541,-0.308638795020976,
0.862505527716294));
#23199=CARTESIAN_POINT('Ctrl Pts',(0.680463863683392,-0.308638795020976,
0.894757676234429));
#23200=CARTESIAN_POINT('Ctrl Pts',(0.657923009631182,-0.305251990234488,
0.91149460735272));
#23201=CARTESIAN_POINT('Ctrl Pts',(0.613307674922609,-0.290879136862659,
0.942092777160053));
#23202=CARTESIAN_POINT('Ctrl Pts',(0.591247219971725,-0.279889827963178,
0.955972930713954));
#23203=CARTESIAN_POINT('Ctrl Pts',(0.548158511259202,-0.251265615809407,
0.981446681891443));
#23204=CARTESIAN_POINT('Ctrl Pts',(0.522002043615455,-0.227269801620063,
0.995447160474328));
#23205=CARTESIAN_POINT('Ctrl Pts',(0.481944444320713,-0.177024326825049,
1.01550068154148));
#23206=CARTESIAN_POINT('Ctrl Pts',(0.463236132117164,-0.14429930310074,
1.0239876538093));
#23207=CARTESIAN_POINT('Ctrl Pts',(0.445111721969657,-0.0928409665394226,
1.03192403056628));
#23208=CARTESIAN_POINT('Ctrl Pts',(0.440685038163619,-0.0762225747374254,
1.03380912944435));
#23209=CARTESIAN_POINT('Ctrl Pts',(0.437601487681056,-0.05953,1.03511272300331));
#23210=CARTESIAN_POINT('Origin',(0.685838782044607,-0.05953,0.860014630714833));
#23211=CARTESIAN_POINT('Origin',(0.,-0.208355,0.));
#23212=CARTESIAN_POINT('',(0.0548532617164168,-0.05953,1.12247250791415));
#23213=CARTESIAN_POINT('Origin',(0.,-0.05953,0.));
#23214=CARTESIAN_POINT('',(-0.536443649899848,-0.05953,0.987512846410683));
#23215=CARTESIAN_POINT('Ctrl Pts',(0.0548532617164173,-0.0595300000000001,
1.12247250791414));
#23216=CARTESIAN_POINT('Ctrl Pts',(0.05150947068137,-0.0762225747374254,
1.12263591311425));
#23217=CARTESIAN_POINT('Ctrl Pts',(0.0467032526342597,-0.0928409665394227,
1.12285816383385));
#23218=CARTESIAN_POINT('Ctrl Pts',(0.0269302585198975,-0.144299303100741,
1.12357162229597));
#23219=CARTESIAN_POINT('Ctrl Pts',(0.006392292392153,-0.177024326825049,
1.12404235695137));
#23220=CARTESIAN_POINT('Ctrl Pts',(-0.0383992541984087,-0.227269801620063,
1.12335509974011));
#23221=CARTESIAN_POINT('Ctrl Pts',(-0.0680399972366993,-0.251265615809407,
1.12208997038458));
#23222=CARTESIAN_POINT('Ctrl Pts',(-0.117914228755037,-0.279889827963178,
1.1178344036749));
#23223=CARTESIAN_POINT('Ctrl Pts',(-0.14381238480104,-0.290879136862659,
1.11490049012186));
#23224=CARTESIAN_POINT('Ctrl Pts',(-0.19728546073067,-0.305251990234488,
1.10669035995599));
#23225=CARTESIAN_POINT('Ctrl Pts',(-0.224855950742601,-0.308638795020976,
1.10139101611326));
#23226=CARTESIAN_POINT('Ctrl Pts',(-0.275287440920027,-0.308638795020976,
1.0898803575765));
#23227=CARTESIAN_POINT('Ctrl Pts',(-0.302426893214945,-0.305251990234488,
1.08269251410343));
#23228=CARTESIAN_POINT('Ctrl Pts',(-0.35416671187353,-0.290879136862659,
1.06688848765783));
#23229=CARTESIAN_POINT('Ctrl Pts',(-0.3787731215897,-0.279889827963178,
1.05829506364875));
#23230=CARTESIAN_POINT('Ctrl Pts',(-0.425554672694338,-0.251265615809407,
1.04048957871266));
#23231=CARTESIAN_POINT('Ctrl Pts',(-0.452808978448581,-0.227269801620063,
1.02876878445619));
#23232=CARTESIAN_POINT('Ctrl Pts',(-0.493462957200432,-0.177024326825049,
1.0099536580922));
#23233=CARTESIAN_POINT('Ctrl Pts',(-0.511762781179148,-0.14429930310074,
1.00061845128527));
#23234=CARTESIAN_POINT('Ctrl Pts',(-0.529268075276157,-0.0928409665394226,
0.991396466802468));
#23235=CARTESIAN_POINT('Ctrl Pts',(-0.533501897135713,-0.0762225747374254,
0.989110885965947));
#23236=CARTESIAN_POINT('Ctrl Pts',(-0.536443649899848,-0.0595300000000001,
0.987512846410683));
#23237=CARTESIAN_POINT('',(-0.843383895613249,-0.05953,0.742736168477219));
#23238=CARTESIAN_POINT('Origin',(0.,-0.05953,0.));
#23239=CARTESIAN_POINT('',(-1.10653577764992,-0.05953,0.196295654879792));
#23240=CARTESIAN_POINT('Ctrl Pts',(-0.843383895613249,-0.0595300000000001,
0.742736168477219));
#23241=CARTESIAN_POINT('Ctrl Pts',(-0.84559647055299,-0.0762225747374255,
0.740223768851062));
#23242=CARTESIAN_POINT('Ctrl Pts',(-0.848766861100456,-0.0928409665394227,
0.736604687327351));
#23243=CARTESIAN_POINT('Ctrl Pts',(-0.861652925570091,-0.144299303100741,
0.721590372101268));
#23244=CARTESIAN_POINT('Ctrl Pts',(-0.87482617317514,-0.177024326825049,
0.705826641853758));
#23245=CARTESIAN_POINT('Ctrl Pts',(-0.902215926359523,-0.227269801620063,
0.670378702718353));
#23246=CARTESIAN_POINT('Ctrl Pts',(-0.919707509403859,-0.251265615809407,
0.646415841396062));
#23247=CARTESIAN_POINT('Ctrl Pts',(-0.947476448101718,-0.279889827963178,
0.604769294586516));
#23248=CARTESIAN_POINT('Ctrl Pts',(-0.961329858300736,-0.290879136862659,
0.582692035672022));
#23249=CARTESIAN_POINT('Ctrl Pts',(-0.988250837578047,-0.305251990234488,
0.535766169015486));
#23250=CARTESIAN_POINT('Ctrl Pts',(-1.00129756308006,-0.308638795020976,
0.510906605094603));
#23251=CARTESIAN_POINT('Ctrl Pts',(-1.02374168767024,-0.308638795020976,
0.46430090015576));
#23252=CARTESIAN_POINT('Ctrl Pts',(-1.03504317708586,-0.305251990234488,
0.438600874831839));
#23253=CARTESIAN_POINT('Ctrl Pts',(-1.05494634094458,-0.290879136862659,
0.388295406390235));
#23254=CARTESIAN_POINT('Ctrl Pts',(-1.06356957703048,-0.279889827963178,
0.363699428370917));
#23255=CARTESIAN_POINT('Ctrl Pts',(-1.0788165083757,-0.251265615809407,
0.316022600643821));
#23256=CARTESIAN_POINT('Ctrl Pts',(-1.08664560412098,-0.227269801620063,
0.287406530683752));
#23257=CARTESIAN_POINT('Ctrl Pts',(-1.09728268713976,-0.177024326825049,
0.243890930799337));
#23258=CARTESIAN_POINT('Ctrl Pts',(-1.10139388218929,-0.144299303100741,
0.22376314604679));
#23259=CARTESIAN_POINT('Ctrl Pts',(-1.10509821673782,-0.0928409665394227,
0.204327142733961));
#23260=CARTESIAN_POINT('Ctrl Pts',(-1.10595102243643,-0.0762225747374254,
0.199591971170104));
#23261=CARTESIAN_POINT('Ctrl Pts',(-1.10653577764992,-0.0595300000000001,
0.196295654879792));
#23262=CARTESIAN_POINT('',(-1.123812,-0.05953,1.37627276864339E-16));
#23263=CARTESIAN_POINT('Origin',(0.,-0.05953,0.));
#23264=CARTESIAN_POINT('',(-1.123812,-0.35718,1.37627276864339E-16));
#23265=CARTESIAN_POINT('',(-1.123812,-0.208355,1.37627276864339E-16));
#23266=CARTESIAN_POINT('Origin',(0.,-0.35718,0.));
#23267=CARTESIAN_POINT('',(-1.10653577764992,-0.05953,-0.196295654879793));
#23268=CARTESIAN_POINT('Origin',(0.,-0.05953,0.));
#23269=CARTESIAN_POINT('',(-0.843383895613249,-0.05953,-0.742736168477219));
#23270=CARTESIAN_POINT('Ctrl Pts',(-1.10653577764992,-0.0595300000000001,
-0.196295654879792));
#23271=CARTESIAN_POINT('Ctrl Pts',(-1.10595102243643,-0.0762225747374255,
-0.199591971170104));
#23272=CARTESIAN_POINT('Ctrl Pts',(-1.10509821673782,-0.0928409665394228,
-0.204327142733962));
#23273=CARTESIAN_POINT('Ctrl Pts',(-1.10139388218929,-0.144299303100741,
-0.22376314604679));
#23274=CARTESIAN_POINT('Ctrl Pts',(-1.09728268713976,-0.177024326825049,
-0.243890930799338));
#23275=CARTESIAN_POINT('Ctrl Pts',(-1.08664560412098,-0.227269801620063,
-0.287406530683753));
#23276=CARTESIAN_POINT('Ctrl Pts',(-1.0788165083757,-0.251265615809407,
-0.316022600643821));
#23277=CARTESIAN_POINT('Ctrl Pts',(-1.06356957703048,-0.279889827963178,
-0.363699428370918));
#23278=CARTESIAN_POINT('Ctrl Pts',(-1.05494634094458,-0.290879136862659,
-0.388295406390235));
#23279=CARTESIAN_POINT('Ctrl Pts',(-1.03504317708586,-0.305251990234488,
-0.438600874831839));
#23280=CARTESIAN_POINT('Ctrl Pts',(-1.02374168767024,-0.308638795020976,
-0.46430090015576));
#23281=CARTESIAN_POINT('Ctrl Pts',(-1.00129756308006,-0.308638795020976,
-0.510906605094603));
#23282=CARTESIAN_POINT('Ctrl Pts',(-0.988250837578047,-0.305251990234488,
-0.535766169015486));
#23283=CARTESIAN_POINT('Ctrl Pts',(-0.961329858300736,-0.290879136862659,
-0.582692035672022));
#23284=CARTESIAN_POINT('Ctrl Pts',(-0.947476448101718,-0.279889827963178,
-0.604769294586516));
#23285=CARTESIAN_POINT('Ctrl Pts',(-0.919707509403859,-0.251265615809407,
-0.646415841396062));
#23286=CARTESIAN_POINT('Ctrl Pts',(-0.902215926359523,-0.227269801620064,
-0.670378702718353));
#23287=CARTESIAN_POINT('Ctrl Pts',(-0.87482617317514,-0.177024326825049,
-0.705826641853758));
#23288=CARTESIAN_POINT('Ctrl Pts',(-0.861652925570091,-0.144299303100741,
-0.721590372101268));
#23289=CARTESIAN_POINT('Ctrl Pts',(-0.848766861100456,-0.0928409665394229,
-0.736604687327351));
#23290=CARTESIAN_POINT('Ctrl Pts',(-0.84559647055299,-0.0762225747374255,
-0.740223768851063));
#23291=CARTESIAN_POINT('Ctrl Pts',(-0.843383895613249,-0.0595300000000001,
-0.742736168477219));
#23292=CARTESIAN_POINT('',(-0.536443649899847,-0.05953,-0.987512846410683));
#23293=CARTESIAN_POINT('Origin',(0.,-0.05953,0.));
#23294=CARTESIAN_POINT('',(0.0548532617164172,-0.05953,-1.12247250791415));
#23295=CARTESIAN_POINT('Ctrl Pts',(-0.536443649899848,-0.0595300000000001,
-0.987512846410683));
#23296=CARTESIAN_POINT('Ctrl Pts',(-0.533501897135712,-0.0762225747374254,
-0.989110885965947));
#23297=CARTESIAN_POINT('Ctrl Pts',(-0.529268075276156,-0.0928409665394227,
-0.991396466802469));
#23298=CARTESIAN_POINT('Ctrl Pts',(-0.511762781179147,-0.144299303100741,
-1.00061845128527));
#23299=CARTESIAN_POINT('Ctrl Pts',(-0.493462957200432,-0.177024326825049,
-1.0099536580922));
#23300=CARTESIAN_POINT('Ctrl Pts',(-0.45280897844858,-0.227269801620063,
-1.02876878445619));
#23301=CARTESIAN_POINT('Ctrl Pts',(-0.425554672694337,-0.251265615809407,
-1.04048957871266));
#23302=CARTESIAN_POINT('Ctrl Pts',(-0.3787731215897,-0.279889827963178,
-1.05829506364875));
#23303=CARTESIAN_POINT('Ctrl Pts',(-0.354166711873529,-0.290879136862659,
-1.06688848765783));
#23304=CARTESIAN_POINT('Ctrl Pts',(-0.302426893214944,-0.305251990234488,
-1.08269251410343));
#23305=CARTESIAN_POINT('Ctrl Pts',(-0.275287440920027,-0.308638795020976,
-1.0898803575765));
#23306=CARTESIAN_POINT('Ctrl Pts',(-0.224855950742601,-0.308638795020976,
-1.10139101611326));
#23307=CARTESIAN_POINT('Ctrl Pts',(-0.19728546073067,-0.305251990234488,
-1.10669035995599));
#23308=CARTESIAN_POINT('Ctrl Pts',(-0.143812384801039,-0.290879136862659,
-1.11490049012186));
#23309=CARTESIAN_POINT('Ctrl Pts',(-0.117914228755037,-0.279889827963178,
-1.1178344036749));
#23310=CARTESIAN_POINT('Ctrl Pts',(-0.0680399972366989,-0.251265615809407,
-1.12208997038458));
#23311=CARTESIAN_POINT('Ctrl Pts',(-0.0383992541984084,-0.227269801620063,
-1.12335509974011));
#23312=CARTESIAN_POINT('Ctrl Pts',(0.00639229239215326,-0.177024326825049,
-1.12404235695137));
#23313=CARTESIAN_POINT('Ctrl Pts',(0.0269302585198977,-0.144299303100741,
-1.12357162229597));
#23314=CARTESIAN_POINT('Ctrl Pts',(0.04670325263426,-0.0928409665394228,
-1.12285816383385));
#23315=CARTESIAN_POINT('Ctrl Pts',(0.0515094706813703,-0.0762225747374255,
-1.12263591311425));
#23316=CARTESIAN_POINT('Ctrl Pts',(0.0548532617164176,-0.0595300000000001,
-1.12247250791414));
#23317=CARTESIAN_POINT('',(0.437601487681057,-0.05953,-1.03511272300331));
#23318=CARTESIAN_POINT('Origin',(0.,-0.05953,0.));
#23319=CARTESIAN_POINT('',(0.911784794170997,-0.05953,-0.656964154625313));
#23320=CARTESIAN_POINT('Ctrl Pts',(0.437601487681056,-0.0595300000000001,
-1.03511272300331));
#23321=CARTESIAN_POINT('Ctrl Pts',(0.440685038163619,-0.0762225747374255,
-1.03380912944435));
#23322=CARTESIAN_POINT('Ctrl Pts',(0.445111721969657,-0.0928409665394228,
-1.03192403056628));
#23323=CARTESIAN_POINT('Ctrl Pts',(0.463236132117164,-0.144299303100741,
-1.0239876538093));
#23324=CARTESIAN_POINT('Ctrl Pts',(0.481944444320713,-0.177024326825049,
-1.01550068154148));
#23325=CARTESIAN_POINT('Ctrl Pts',(0.522002043615455,-0.227269801620064,
-0.995447160474328));
#23326=CARTESIAN_POINT('Ctrl Pts',(0.548158511259203,-0.251265615809407,
-0.981446681891443));
#23327=CARTESIAN_POINT('Ctrl Pts',(0.591247219971725,-0.279889827963178,
-0.955972930713954));
#23328=CARTESIAN_POINT('Ctrl Pts',(0.613307674922609,-0.290879136862659,
-0.942092777160053));
#23329=CARTESIAN_POINT('Ctrl Pts',(0.657923009631182,-0.305251990234487,
-0.91149460735272));
#23330=CARTESIAN_POINT('Ctrl Pts',(0.680463863683393,-0.308638795020976,
-0.894757676234429));
#23331=CARTESIAN_POINT('Ctrl Pts',(0.720906778729542,-0.308638795020976,
-0.862505527716294));
#23332=CARTESIAN_POINT('Ctrl Pts',(0.742239891936899,-0.305251990234488,
-0.844254137480381));
#23333=CARTESIAN_POINT('Ctrl Pts',(0.781998747691872,-0.290879136862659,
-0.80756613568454));
#23334=CARTESIAN_POINT('Ctrl Pts',(0.800439809856112,-0.279889827963178,
-0.789147407129765));
#23335=CARTESIAN_POINT('Ctrl Pts',(0.834863020612702,-0.251265615809407,
-0.752807465209441));
#23336=CARTESIAN_POINT('Ctrl Pts',(0.854332839576145,-0.227269801620064,
-0.73042219438957));
#23337=CARTESIAN_POINT('Ctrl Pts',(0.882797231409153,-0.177024326825049,
-0.695831250979106));
#23338=CARTESIAN_POINT('Ctrl Pts',(0.895234408667242,-0.144299303100741,
-0.679480524217551));
#23339=CARTESIAN_POINT('Ctrl Pts',(0.907004864562642,-0.0928409665394228,
-0.663576540841106));
#23340=CARTESIAN_POINT('Ctrl Pts',(0.909827729890942,-0.0762225747374256,
-0.659680317203144));
#23341=CARTESIAN_POINT('Ctrl Pts',(0.911784794170998,-0.0595300000000001,
-0.656964154625312));
#23342=CARTESIAN_POINT('',(1.08212377959455,-0.05953,-0.303251606722892));
#23343=CARTESIAN_POINT('Origin',(0.,-0.05953,0.));
#23344=CARTESIAN_POINT('',(1.08212377959455,-0.05953,0.303251606722892));
#23345=CARTESIAN_POINT('Ctrl Pts',(1.08212377959455,-0.0595300000000001,
-0.303251606722892));
#23346=CARTESIAN_POINT('Ctrl Pts',(1.0830271513892,-0.0762225747374255,
-0.300028012588062));
#23347=CARTESIAN_POINT('Ctrl Pts',(1.08431331394788,-0.0928409665394228,
-0.2953917518996));
#23348=CARTESIAN_POINT('Ctrl Pts',(1.08940878963422,-0.144299303100741,
-0.276273267473431));
#23349=CARTESIAN_POINT('Ctrl Pts',(1.09443784939331,-0.177024326825049,
-0.256354979351213));
#23350=CARTESIAN_POINT('Ctrl Pts',(1.10373487993589,-0.227269801620064,
-0.212533521233765));
#23351=CARTESIAN_POINT('Ctrl Pts',(1.10909715583869,-0.251265615809407,
-0.183354415742157));
#23352=CARTESIAN_POINT('Ctrl Pts',(1.1160463456491,-0.279889827963178,-0.133783682657561));
#23353=CARTESIAN_POINT('Ctrl Pts',(1.11894887330541,-0.290879136862659,
-0.107881990270302));
#23354=CARTESIAN_POINT('Ctrl Pts',(1.12284346704144,-0.305251990234488,
-0.0539226701638766));
#23355=CARTESIAN_POINT('Ctrl Pts',(1.123812,-0.308638795020976,-0.025864214957475));
#23356=CARTESIAN_POINT('Ctrl Pts',(1.123812,-0.308638795020976,0.025864214957475));
#23357=CARTESIAN_POINT('Ctrl Pts',(1.12284346704144,-0.305251990234488,
0.0539226701638766));
#23358=CARTESIAN_POINT('Ctrl Pts',(1.11894887330541,-0.290879136862659,
0.107881990270302));
#23359=CARTESIAN_POINT('Ctrl Pts',(1.1160463456491,-0.279889827963178,0.133783682657561));
#23360=CARTESIAN_POINT('Ctrl Pts',(1.10909715583869,-0.251265615809407,
0.183354415742157));
#23361=CARTESIAN_POINT('Ctrl Pts',(1.10373487993589,-0.227269801620064,
0.212533521233765));
#23362=CARTESIAN_POINT('Ctrl Pts',(1.09443784939331,-0.177024326825049,
0.256354979351213));
#23363=CARTESIAN_POINT('Ctrl Pts',(1.08940878963422,-0.144299303100741,
0.276273267473431));
#23364=CARTESIAN_POINT('Ctrl Pts',(1.08431331394788,-0.0928409665394228,
0.2953917518996));
#23365=CARTESIAN_POINT('Ctrl Pts',(1.0830271513892,-0.0762225747374255,
0.300028012588062));
#23366=CARTESIAN_POINT('Ctrl Pts',(1.08212377959455,-0.0595300000000001,
0.303251606722892));
#23367=CARTESIAN_POINT('Origin',(0.,-0.05953,0.));
#23368=CARTESIAN_POINT('Origin',(0.,-0.05953,0.));
#23369=CARTESIAN_POINT('',(0.0589974094846122,-0.05953,1.07456964270265));
#23370=CARTESIAN_POINT('Origin',(0.,-0.05953,0.));
#23371=CARTESIAN_POINT('Origin',(-0.244773027351946,-0.05953,1.07242070340001));
#23372=CARTESIAN_POINT('Origin',(-0.244773027351946,0.,1.07242070340001));
#23373=CARTESIAN_POINT('',(-0.519393123750572,-0.05953,0.942555777842682));
#23374=CARTESIAN_POINT('Ctrl Pts',(-0.519393123750572,-0.05953,0.942555777842682));
#23375=CARTESIAN_POINT('Ctrl Pts',(-0.513714466572041,-0.0925528133349865,
0.945684988399766));
#23376=CARTESIAN_POINT('Ctrl Pts',(-0.503136848051455,-0.124911173756694,
0.951483858396181));
#23377=CARTESIAN_POINT('Ctrl Pts',(-0.47593627990192,-0.177924977804098,
0.965323333309091));
#23378=CARTESIAN_POINT('Ctrl Pts',(-0.460931856495794,-0.199697230012983,
0.972669835243841));
#23379=CARTESIAN_POINT('Ctrl Pts',(-0.426157505475872,-0.237895043532788,
0.988400002689705));
#23380=CARTESIAN_POINT('Ctrl Pts',(-0.406380688682952,-0.254319232363049,
0.996771768218699));
#23381=CARTESIAN_POINT('Ctrl Pts',(-0.364750145543744,-0.28018331644634,
1.01272583306292));
#23382=CARTESIAN_POINT('Ctrl Pts',(-0.340838910881557,-0.29104845371857,
1.02112815447116));
#23383=CARTESIAN_POINT('Ctrl Pts',(-0.290495481564827,-0.30527573347708,
1.036574285215));
#23384=CARTESIAN_POINT('Ctrl Pts',(-0.264056468041074,-0.308638795020976,
1.04359501395068));
#23385=CARTESIAN_POINT('Ctrl Pts',(-0.214892249704082,-0.308638795020976,
1.05481642595959));
#23386=CARTESIAN_POINT('Ctrl Pts',(-0.188025341585962,-0.30527573347708,
1.05996242598502));
#23387=CARTESIAN_POINT('Ctrl Pts',(-0.135965654106109,-0.29104845371857,
1.06788913840721));
#23388=CARTESIAN_POINT('Ctrl Pts',(-0.110776745452494,-0.28018331644634,
1.07069360430242));
#23389=CARTESIAN_POINT('Ctrl Pts',(-0.0663467128214646,-0.254319232363049,
1.07438230428002));
#23390=CARTESIAN_POINT('Ctrl Pts',(-0.0448960436540983,-0.237895043532788,
1.07542044338697));
#23391=CARTESIAN_POINT('Ctrl Pts',(-0.00674037211528124,-0.199697230012983,
1.07633607767727));
#23392=CARTESIAN_POINT('Ctrl Pts',(0.00996567398334777,-0.177924977804098,
1.07622728347683));
#23393=CARTESIAN_POINT('Ctrl Pts',(0.0404772621979741,-0.124911173756694,
1.07556023164702));
#23394=CARTESIAN_POINT('Ctrl Pts',(0.0525234025782719,-0.0925528133349865,
1.07492508698591));
#23395=CARTESIAN_POINT('Ctrl Pts',(0.0589974094846124,-0.05953,1.07456964270265));
#23396=CARTESIAN_POINT('Origin',(-0.244773027351946,-0.05953,1.07242070340001));
#23397=CARTESIAN_POINT('Origin',(0.,-0.05953,0.));
#23398=CARTESIAN_POINT('',(-0.803348093619616,-0.05953,0.716109245731214));
#23399=CARTESIAN_POINT('Origin',(0.,-0.05953,0.));
#23400=CARTESIAN_POINT('Origin',(-0.991065754692661,-0.05953,0.477272113029314));
#23401=CARTESIAN_POINT('Origin',(-0.991065754692661,0.,0.477272113029314));
#23402=CARTESIAN_POINT('',(-1.06075609691358,-0.05953,0.181596019242328));
#23403=CARTESIAN_POINT('Ctrl Pts',(-1.06075609691358,-0.05953,0.181596019242328));
#23404=CARTESIAN_POINT('Ctrl Pts',(-1.05966202740332,-0.0925528133349865,
0.187986803072856));
#23405=CARTESIAN_POINT('Ctrl Pts',(-1.05760072925372,-0.124911173756694,
0.199872254546857));
#23406=CARTESIAN_POINT('Ctrl Pts',(-1.05146158959546,-0.177924977804098,
0.22976728653846));
#23407=CARTESIAN_POINT('Ctrl Pts',(-1.04785021111757,-0.199697230012983,
0.246078686169301));
#23408=CARTESIAN_POINT('Ctrl Pts',(-1.03846709802406,-0.237895043532788,
0.283073967563097));
#23409=CARTESIAN_POINT('Ctrl Pts',(-1.03268176429485,-0.254319232363049,
0.303755815985685));
#23410=CARTESIAN_POINT('Ctrl Pts',(-1.01919893537026,-0.28018331644634,
0.346251081972725));
#23411=CARTESIAN_POINT('Ctrl Pts',(-1.01085972381132,-0.29104845371857,
0.370184399726282));
#23412=CARTESIAN_POINT('Ctrl Pts',(-0.99154738033959,-0.30527573347708,
0.419174982698463));
#23413=CARTESIAN_POINT('Ctrl Pts',(-0.980551951791748,-0.308638795020976,
0.444223188605045));
#23414=CARTESIAN_POINT('Ctrl Pts',(-0.958671816228589,-0.308638795020976,
0.489657758261848));
#23415=CARTESIAN_POINT('Ctrl Pts',(-0.945943877838127,-0.30527573347708,
0.51387163140139));
#23416=CARTESIAN_POINT('Ctrl Pts',(-0.91968254693063,-0.29104845371857,
0.559515758398093));
#23417=CARTESIAN_POINT('Ctrl Pts',(-0.906170138993533,-0.28018331644634,
0.580957796077825));
#23418=CARTESIAN_POINT('Ctrl Pts',(-0.8813524085237,-0.254319232363049,
0.617994461173994));
#23419=CARTESIAN_POINT('Ctrl Pts',(-0.868789784891799,-0.237895043532788,
0.635412538795143));
#23420=CARTESIAN_POINT('Ctrl Pts',(-0.845715984518854,-0.199697230012983,
0.66581473268113));
#23421=CARTESIAN_POINT('Ctrl Pts',(-0.835214876415962,-0.177924977804098,
0.678808213394124));
#23422=CARTESIAN_POINT('Ctrl Pts',(-0.815669690204649,-0.124911173756694,
0.702247233627224));
#23423=CARTESIAN_POINT('Ctrl Pts',(-0.807662468433796,-0.0925528133349865,
0.711269279199861));
#23424=CARTESIAN_POINT('Ctrl Pts',(-0.803348093619616,-0.05953,0.716109245731214));
#23425=CARTESIAN_POINT('Origin',(-0.991065754692661,-0.05953,0.477272113029314));
#23426=CARTESIAN_POINT('Origin',(0.,-0.05953,0.));
#23427=CARTESIAN_POINT('',(-1.076188,-0.05953,1.31795018948079E-16));
#23428=CARTESIAN_POINT('Origin',(0.,-0.05953,0.));
#23429=CARTESIAN_POINT('',(-1.06075609691358,-0.05953,-0.181596019242328));
#23430=CARTESIAN_POINT('Origin',(0.,-0.05953,0.));
#23431=CARTESIAN_POINT('Origin',(-0.991065754692661,-0.05953,-0.477272113029314));
#23432=CARTESIAN_POINT('Origin',(-0.991065754692661,0.,-0.477272113029314));
#23433=CARTESIAN_POINT('',(-0.803348093619616,-0.05953,-0.716109245731215));
#23434=CARTESIAN_POINT('Ctrl Pts',(-0.803348093619616,-0.05953,-0.716109245731215));
#23435=CARTESIAN_POINT('Ctrl Pts',(-0.807662468433795,-0.0925528133349865,
-0.711269279199862));
#23436=CARTESIAN_POINT('Ctrl Pts',(-0.815669690204649,-0.124911173756694,
-0.702247233627224));
#23437=CARTESIAN_POINT('Ctrl Pts',(-0.835214876415962,-0.177924977804098,
-0.678808213394124));
#23438=CARTESIAN_POINT('Ctrl Pts',(-0.845715984518854,-0.199697230012983,
-0.66581473268113));
#23439=CARTESIAN_POINT('Ctrl Pts',(-0.868789784891799,-0.237895043532788,
-0.635412538795143));
#23440=CARTESIAN_POINT('Ctrl Pts',(-0.8813524085237,-0.254319232363049,
-0.617994461173994));
#23441=CARTESIAN_POINT('Ctrl Pts',(-0.906170138993533,-0.28018331644634,
-0.580957796077826));
#23442=CARTESIAN_POINT('Ctrl Pts',(-0.91968254693063,-0.29104845371857,
-0.559515758398093));
#23443=CARTESIAN_POINT('Ctrl Pts',(-0.945943877838127,-0.30527573347708,
-0.51387163140139));
#23444=CARTESIAN_POINT('Ctrl Pts',(-0.958671816228589,-0.308638795020976,
-0.489657758261848));
#23445=CARTESIAN_POINT('Ctrl Pts',(-0.980551951791748,-0.308638795020976,
-0.444223188605045));
#23446=CARTESIAN_POINT('Ctrl Pts',(-0.99154738033959,-0.30527573347708,
-0.419174982698463));
#23447=CARTESIAN_POINT('Ctrl Pts',(-1.01085972381132,-0.29104845371857,
-0.370184399726282));
#23448=CARTESIAN_POINT('Ctrl Pts',(-1.01919893537026,-0.28018331644634,
-0.346251081972725));
#23449=CARTESIAN_POINT('Ctrl Pts',(-1.03268176429485,-0.254319232363049,
-0.303755815985685));
#23450=CARTESIAN_POINT('Ctrl Pts',(-1.03846709802406,-0.237895043532788,
-0.283073967563097));
#23451=CARTESIAN_POINT('Ctrl Pts',(-1.04785021111757,-0.199697230012983,
-0.246078686169302));
#23452=CARTESIAN_POINT('Ctrl Pts',(-1.05146158959546,-0.177924977804098,
-0.229767286538461));
#23453=CARTESIAN_POINT('Ctrl Pts',(-1.05760072925372,-0.124911173756694,
-0.199872254546858));
#23454=CARTESIAN_POINT('Ctrl Pts',(-1.05966202740332,-0.0925528133349864,
-0.187986803072857));
#23455=CARTESIAN_POINT('Ctrl Pts',(-1.06075609691358,-0.05953,-0.181596019242328));
#23456=CARTESIAN_POINT('Origin',(-0.991065754692661,-0.05953,-0.477272113029314));
#23457=CARTESIAN_POINT('Origin',(0.,-0.05953,0.));
#23458=CARTESIAN_POINT('',(-0.519393123750572,-0.05953,-0.942555777842682));
#23459=CARTESIAN_POINT('Origin',(0.,-0.05953,0.));
#23460=CARTESIAN_POINT('Origin',(-0.244773027351946,-0.05953,-1.07242070340001));
#23461=CARTESIAN_POINT('Origin',(-0.244773027351946,0.,-1.07242070340001));
#23462=CARTESIAN_POINT('',(0.0589974094846125,-0.05953,-1.07456964270265));
#23463=CARTESIAN_POINT('Ctrl Pts',(0.0589974094846127,-0.05953,-1.07456964270265));
#23464=CARTESIAN_POINT('Ctrl Pts',(0.0525234025782722,-0.0925528133349865,
-1.07492508698591));
#23465=CARTESIAN_POINT('Ctrl Pts',(0.0404772621979744,-0.124911173756694,
-1.07556023164702));
#23466=CARTESIAN_POINT('Ctrl Pts',(0.0099656739833481,-0.177924977804098,
-1.07622728347683));
#23467=CARTESIAN_POINT('Ctrl Pts',(-0.00674037211528096,-0.199697230012983,
-1.07633607767727));
#23468=CARTESIAN_POINT('Ctrl Pts',(-0.044896043654098,-0.237895043532788,
-1.07542044338697));
#23469=CARTESIAN_POINT('Ctrl Pts',(-0.0663467128214644,-0.254319232363049,
-1.07438230428002));
#23470=CARTESIAN_POINT('Ctrl Pts',(-0.110776745452493,-0.28018331644634,
-1.07069360430242));
#23471=CARTESIAN_POINT('Ctrl Pts',(-0.135965654106109,-0.29104845371857,
-1.06788913840721));
#23472=CARTESIAN_POINT('Ctrl Pts',(-0.188025341585962,-0.30527573347708,
-1.05996242598502));
#23473=CARTESIAN_POINT('Ctrl Pts',(-0.214892249704082,-0.308638795020976,
-1.05481642595959));
#23474=CARTESIAN_POINT('Ctrl Pts',(-0.264056468041074,-0.308638795020976,
-1.04359501395068));
#23475=CARTESIAN_POINT('Ctrl Pts',(-0.290495481564827,-0.30527573347708,
-1.036574285215));
#23476=CARTESIAN_POINT('Ctrl Pts',(-0.340838910881557,-0.291048453718569,
-1.02112815447116));
#23477=CARTESIAN_POINT('Ctrl Pts',(-0.364750145543744,-0.28018331644634,
-1.01272583306292));
#23478=CARTESIAN_POINT('Ctrl Pts',(-0.406380688682952,-0.254319232363049,
-0.996771768218699));
#23479=CARTESIAN_POINT('Ctrl Pts',(-0.426157505475872,-0.237895043532788,
-0.988400002689705));
#23480=CARTESIAN_POINT('Ctrl Pts',(-0.460931856495794,-0.199697230012983,
-0.972669835243841));
#23481=CARTESIAN_POINT('Ctrl Pts',(-0.475936279901919,-0.177924977804098,
-0.965323333309091));
#23482=CARTESIAN_POINT('Ctrl Pts',(-0.503136848051454,-0.124911173756694,
-0.951483858396181));
#23483=CARTESIAN_POINT('Ctrl Pts',(-0.513714466572041,-0.0925528133349865,
-0.945684988399766));
#23484=CARTESIAN_POINT('Ctrl Pts',(-0.519393123750572,-0.05953,-0.942555777842682));
#23485=CARTESIAN_POINT('Origin',(-0.244773027351946,-0.05953,-1.07242070340001));
#23486=CARTESIAN_POINT('Origin',(0.,-0.05953,0.));
#23487=CARTESIAN_POINT('',(0.413083465285518,-0.05953,-0.993751811093549));
#23488=CARTESIAN_POINT('Origin',(0.,-0.05953,0.));
#23489=CARTESIAN_POINT('Origin',(0.685838782044607,-0.05953,-0.860014630714833));
#23490=CARTESIAN_POINT('Origin',(0.685838782044607,0.,-0.860014630714833));
#23491=CARTESIAN_POINT('',(0.876916659919095,-0.05953,-0.623857181492959));
#23492=CARTESIAN_POINT('Ctrl Pts',(0.876916659919095,-0.05953,-0.623857181492958));
#23493=CARTESIAN_POINT('Ctrl Pts',(0.873158080166742,-0.0925528133349865,
-0.62914037979579));
#23494=CARTESIAN_POINT('Ctrl Pts',(0.866144010579847,-0.124911173756694,
-0.638954437806245));
#23495=CARTESIAN_POINT('Ctrl Pts',(0.847641868610495,-0.177924977804098,
-0.663225258065736));
#23496=CARTESIAN_POINT('Ctrl Pts',(0.837310877969633,-0.199697230012983,
-0.676354402927683));
#23497=CARTESIAN_POINT('Ctrl Pts',(0.81280533416753,-0.237895043532788,
-0.705614819529209));
#23498=CARTESIAN_POINT('Ctrl Pts',(0.798619410861634,-0.254319232363049,
-0.721738358858166));
#23499=CARTESIAN_POINT('Ctrl Pts',(0.768033796848072,-0.28018331644634,
-0.754175290318038));
#23500=CARTESIAN_POINT('Ctrl Pts',(0.750136149454208,-0.29104845371857,
-0.772120216227122));
#23501=CARTESIAN_POINT('Ctrl Pts',(0.711480111898423,-0.30527573347708,
-0.807879894508811));
#23502=CARTESIAN_POINT('Ctrl Pts',(0.690705563850638,-0.308638795020976,
-0.825676810575913));
#23503=CARTESIAN_POINT('Ctrl Pts',(0.651278921914856,-0.308638795020976,
-0.857118508332695));
#23504=CARTESIAN_POINT('Ctrl Pts',(0.629305439856167,-0.30527573347708,
-0.873412008702649));
#23505=CARTESIAN_POINT('Ctrl Pts',(0.585840553788742,-0.29104845371857,
-0.903141581680914));
#23506=CARTESIAN_POINT('Ctrl Pts',(0.564362943424239,-0.28018331644634,
-0.916597376014514));
#23507=CARTESIAN_POINT('Ctrl Pts',(0.525933334162556,-0.254319232363049,
-0.939198248544427));
#23508=CARTESIAN_POINT('Ctrl Pts',(0.507057380724533,-0.237895043532788,
-0.949440676105255));
#23509=CARTESIAN_POINT('Ctrl Pts',(0.473077587363686,-0.199697230012983,
-0.966820759530997));
#23510=CARTESIAN_POINT('Ctrl Pts',(0.457978755888596,-0.177924977804098,
-0.973971221090534));
#23511=CARTESIAN_POINT('Ctrl Pts',(0.430199341854858,-0.124911173756694,
-0.986608710139579));
#23512=CARTESIAN_POINT('Ctrl Pts',(0.419070565453384,-0.0925528133349865,
-0.991263089003441));
#23513=CARTESIAN_POINT('Ctrl Pts',(0.413083465285518,-0.05953,-0.993751811093549));
#23514=CARTESIAN_POINT('Origin',(0.685838782044607,-0.05953,-0.860014630714833));
#23515=CARTESIAN_POINT('Origin',(0.,-0.208355,0.));
#23516=CARTESIAN_POINT('',(-1.076188,-0.35718,1.31795018948079E-16));
#23517=CARTESIAN_POINT('Origin',(0.,-0.35718,0.));
#23518=CARTESIAN_POINT('',(-1.076188,-0.208355,1.31795018948079E-16));
#23519=CARTESIAN_POINT('',(1.03449977959455,-0.05953,0.296632461748266));
#23520=CARTESIAN_POINT('Origin',(0.,-0.05953,0.));
#23521=CARTESIAN_POINT('',(1.03449977959455,-0.05953,-0.296632461748266));
#23522=CARTESIAN_POINT('Ctrl Pts',(1.03449977959455,-0.05953,0.296632461748267));
#23523=CARTESIAN_POINT('Ctrl Pts',(1.03628691421076,-0.0925528133349865,
0.290399865505497));
#23524=CARTESIAN_POINT('Ctrl Pts',(1.03958665287714,-0.124911173756694,
0.278797079997872));
#23525=CARTESIAN_POINT('Ctrl Pts',(1.0470264474309,-0.177924977804098,0.249198913998601));
#23526=CARTESIAN_POINT('Ctrl Pts',(1.05084995891418,-0.199697230012983,
0.232935932341942));
#23527=CARTESIAN_POINT('Ctrl Pts',(1.05844771715377,-0.237895043532788,
0.195533155353269));
#23528=CARTESIAN_POINT('Ctrl Pts',(1.06220882929878,-0.254319232363049,
0.17438929156337));
#23529=CARTESIAN_POINT('Ctrl Pts',(1.06849922508772,-0.28018331644634,0.130252399648131));
#23530=CARTESIAN_POINT('Ctrl Pts',(1.07137013248666,-0.29104845371857,0.105070977154072));
#23531=CARTESIAN_POINT('Ctrl Pts',(1.07522652957392,-0.30527573347708,0.0525526752791107));
#23532=CARTESIAN_POINT('Ctrl Pts',(1.076188,-0.308638795020976,0.025214283908933));
#23533=CARTESIAN_POINT('Ctrl Pts',(1.076188,-0.308638795020976,-0.025214283908933));
#23534=CARTESIAN_POINT('Ctrl Pts',(1.07522652957392,-0.30527573347708,-0.0525526752791107));
#23535=CARTESIAN_POINT('Ctrl Pts',(1.07137013248666,-0.29104845371857,-0.105070977154072));
#23536=CARTESIAN_POINT('Ctrl Pts',(1.06849922508772,-0.28018331644634,-0.130252399648131));
#23537=CARTESIAN_POINT('Ctrl Pts',(1.06220882929878,-0.254319232363049,
-0.17438929156337));
#23538=CARTESIAN_POINT('Ctrl Pts',(1.05844771715377,-0.237895043532788,
-0.195533155353269));
#23539=CARTESIAN_POINT('Ctrl Pts',(1.05084995891418,-0.199697230012983,
-0.232935932341942));
#23540=CARTESIAN_POINT('Ctrl Pts',(1.0470264474309,-0.177924977804098,-0.249198913998601));
#23541=CARTESIAN_POINT('Ctrl Pts',(1.03958665287714,-0.124911173756694,
-0.278797079997872));
#23542=CARTESIAN_POINT('Ctrl Pts',(1.03628691421076,-0.0925528133349865,
-0.290399865505497));
#23543=CARTESIAN_POINT('Ctrl Pts',(1.03449977959455,-0.05953,-0.296632461748267));
#23544=CARTESIAN_POINT('Origin',(0.,-0.05953,0.));
#23545=CARTESIAN_POINT('Origin',(0.,-0.05953,0.));
#23546=CARTESIAN_POINT('Origin',(1.1,-0.05953,0.));
#23547=CARTESIAN_POINT('Origin',(1.1,0.,0.));
#23548=CARTESIAN_POINT('Origin',(1.1,-0.05953,0.));
#23549=CARTESIAN_POINT('Origin',(0.,-0.35718,0.));
#23550=CARTESIAN_POINT('Origin',(0.,-0.05953,0.));
#26956=UNCERTAINTY_MEASURE_WITH_UNIT(LENGTH_MEASURE(0.001),#27070,
'DISTANCE_ACCURACY_VALUE',
'Maximum model space distance between geometric entities at asserted c
onnectivities');
#26992=UNCERTAINTY_MEASURE_WITH_UNIT(LENGTH_MEASURE(0.001),#27070,
'DISTANCE_ACCURACY_VALUE',
'Maximum model space distance between geometric entities at asserted c
onnectivities');
#27033=(
GEOMETRIC_REPRESENTATION_CONTEXT(3)
GLOBAL_UNCERTAINTY_ASSIGNED_CONTEXT((#26956))
GLOBAL_UNIT_ASSIGNED_CONTEXT((#27070,#27072,#27073))
REPRESENTATION_CONTEXT('','3D')
);
#27069=(
GEOMETRIC_REPRESENTATION_CONTEXT(3)
GLOBAL_UNCERTAINTY_ASSIGNED_CONTEXT((#26992))
GLOBAL_UNIT_ASSIGNED_CONTEXT((#27070,#27072,#27073))
REPRESENTATION_CONTEXT('','3D')
);
#27070=(
LENGTH_UNIT()
NAMED_UNIT(*)
SI_UNIT(.CENTI.,.METRE.)
);
#27072=(
NAMED_UNIT(*)
PLANE_ANGLE_UNIT()
SI_UNIT($,.RADIAN.)
);
#27073=(
NAMED_UNIT(*)
SI_UNIT($,.STERADIAN.)
SOLID_ANGLE_UNIT()
);
#27114=SHAPE_DEFINITION_REPRESENTATION(#27195,#27391);
#27195=PRODUCT_DEFINITION_SHAPE('',$,#27468);
#27391=SHAPE_REPRESENTATION('',(#15409),#27033);
#27427=PRODUCT_DEFINITION_CONTEXT('part definition',#27657,'design');
#27468=PRODUCT_DEFINITION('Cage (1)','Cage (1)',#27544,#27427);
#27544=PRODUCT_DEFINITION_FORMATION('',$,#27699);
#27657=APPLICATION_CONTEXT(
'Core Data for Automotive Mechanical Design Process');
#27658=PRODUCT_CONTEXT('part definition',#27657,'mechanical');
#27699=PRODUCT('Cage (1)','Cage (1)','Cage (1)',(#27658));
#27791=COLOUR_RGB('Grey',0.48,0.52,0.57);
#27792=FILL_AREA_STYLE_COLOUR('',#27791);
#27793=FILL_AREA_STYLE('',(#27792));
#27794=SURFACE_STYLE_FILL_AREA(#27793);
#27795=SURFACE_SIDE_STYLE('',(#27794));
#27796=SURFACE_STYLE_USAGE(.BOTH.,#27795);
#27797=PRESENTATION_STYLE_ASSIGNMENT((#27796));
ENDSEC;
END-ISO-10303-21;
